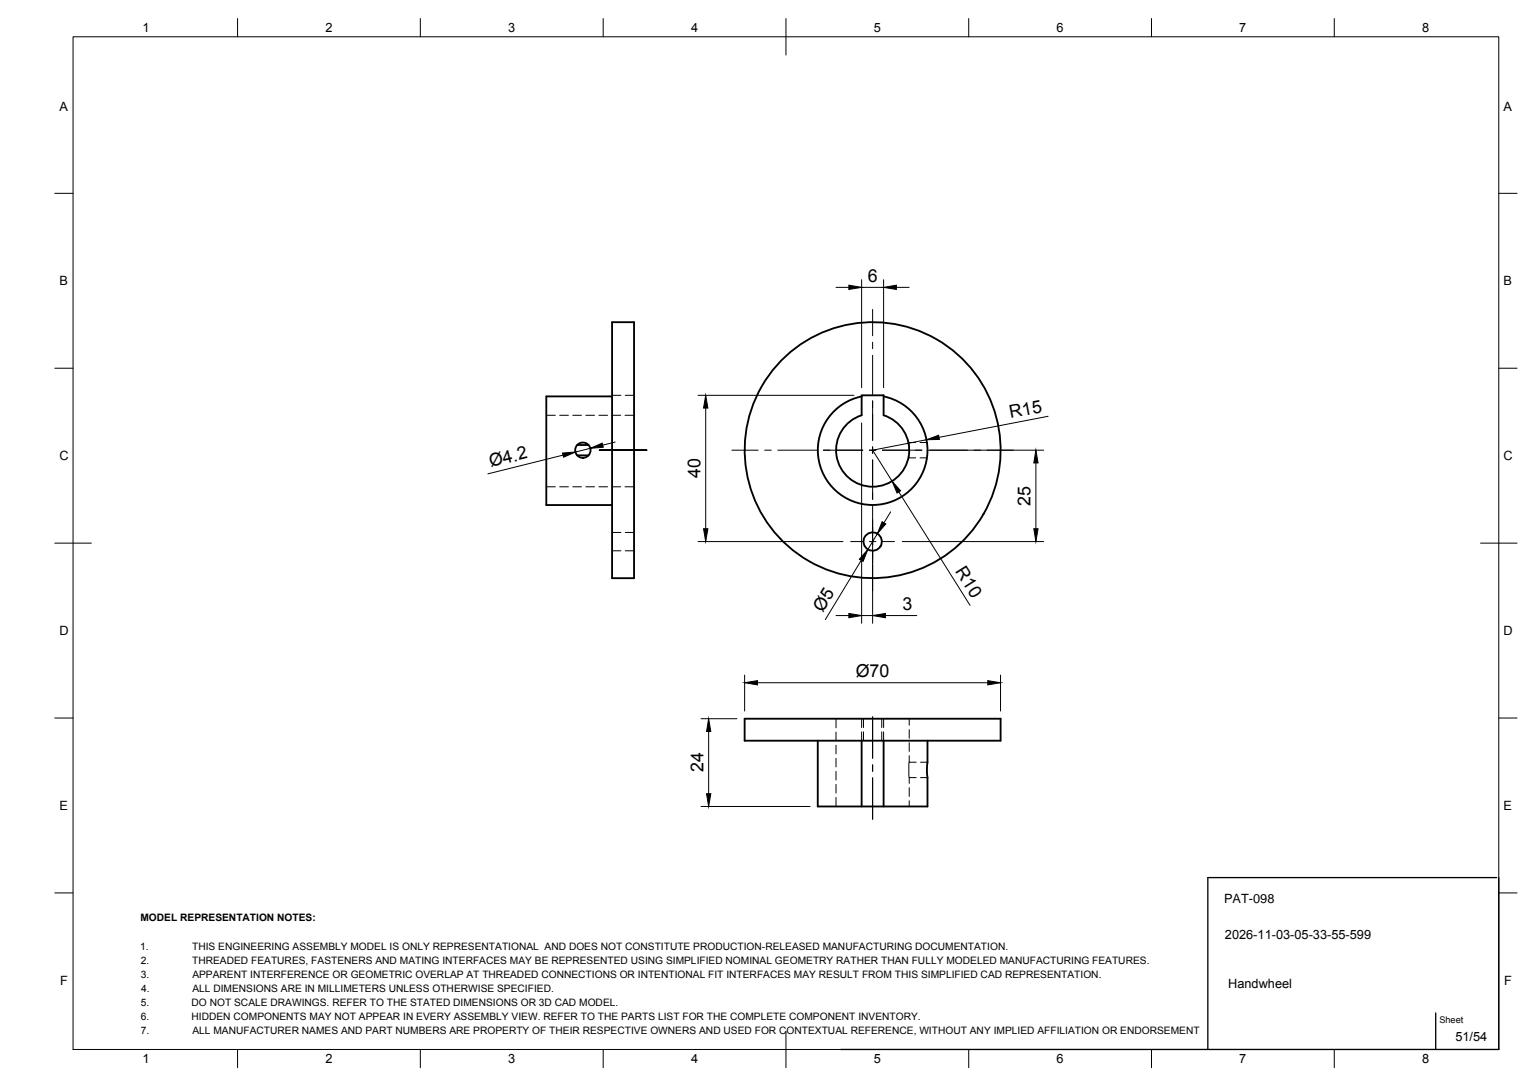
ISO-10303-21;
HEADER;
/* Generated by software containing ST-Developer
 * from STEP Tools, Inc. (www.steptools.com) 
 */

FILE_DESCRIPTION(
/* description */ ('Spring compression tester'),
/* implementation_level */ '2;1');

FILE_NAME(
/* name */ 'Handwheel.step',
/* time_stamp */ '2026-10-28T03:24:11-07:00',
/* author */ (''),
/* organization */ (''),
/* preprocessor_version */ 'ST-DEVELOPER v20.2',
/* originating_system */ 'Autodesk Translation Framework v15.17.0.0',
/* authorisation */ '');

FILE_SCHEMA (('AUTOMOTIVE_DESIGN { 1 0 10303 214 3 1 1 }'));
ENDSEC;

DATA;
#10=MECHANICAL_DESIGN_GEOMETRIC_PRESENTATION_REPRESENTATION('',(#1172),#43521);
#892=B_SPLINE_CURVE_WITH_KNOTS('',3,(#43043,#43044,#43045,#43046,#43047,
#43048),.UNSPECIFIED.,.F.,.F.,(4,2,4),(0.803821788694078,0.872950991853625,
0.952307212900975),.UNSPECIFIED.);
#893=B_SPLINE_CURVE_WITH_KNOTS('',3,(#43051,#43052,#43053,#43054,#43055,
#43056,#43057,#43058,#43059,#43060),.UNSPECIFIED.,.F.,.F.,(4,2,2,2,4),(0.168950313426762,
0.238079516586309,0.317435737633658,0.396791958681008,0.465921161840561),
 .UNSPECIFIED.);
#894=B_SPLINE_CURVE_WITH_KNOTS('',3,(#43061,#43062,#43063,#43064,#43065,
#43066),.UNSPECIFIED.,.F.,.F.,(4,2,4),(0.952307212900975,1.03166343394832,
1.10079263710787),.UNSPECIFIED.);
#895=B_SPLINE_CURVE_WITH_KNOTS('',3,(#43070,#43071,#43072,#43073,#43074,
#43075,#43076,#43077,#43078,#43079),.UNSPECIFIED.,.F.,.F.,(4,2,2,2,4),(0.,
0.0792165807733642,0.158433161546728,0.237648697074572,0.316864232602417),
 .UNSPECIFIED.);
#896=B_SPLINE_CURVE_WITH_KNOTS('',3,(#43080,#43081,#43082,#43083,#43084,
#43085,#43086,#43087,#43088,#43089,#43090,#43091,#43092,#43093,#43094,#43095,
#43096,#43097,#43098,#43099,#43100,#43101,#43102,#43103,#43104,#43105),
 .UNSPECIFIED.,.F.,.F.,(4,2,2,2,2,2,2,2,2,2,2,2,4),(0.316864232602417,0.396079768130261,
0.475295303658105,0.554511884431469,0.633728465204833,0.712945045978197,
0.792161626751562,0.871377162279406,0.95059269780725,1.02980823333509,1.10902376886294,
1.1882403496363,1.26745693040967),.UNSPECIFIED.);
#1037=SHAPE_REPRESENTATION_RELATIONSHIP('SRR','None',#43854,#1097);
#1097=ADVANCED_BREP_SHAPE_REPRESENTATION('',(#1241),#43514);
#1172=STYLED_ITEM('',(#44195),#1241);
#1241=MANIFOLD_SOLID_BREP('Body1',#18615);
#1575=FACE_BOUND('',#4536,.T.);
#1576=FACE_BOUND('',#4537,.T.);
#1577=FACE_BOUND('',#4539,.T.);
#1578=FACE_BOUND('',#4540,.T.);
#1579=FACE_BOUND('',#4543,.T.);
#1580=FACE_BOUND('',#4545,.T.);
#2126=PLANE('',#21081);
#2127=PLANE('',#21085);
#2128=PLANE('',#21086);
#2129=PLANE('',#21087);
#2130=PLANE('',#21088);
#2131=PLANE('',#21089);
#2132=PLANE('',#21092);
#2133=PLANE('',#21100);
#3153=FACE_OUTER_BOUND('',#4528,.T.);
#3154=FACE_OUTER_BOUND('',#4529,.T.);
#3155=FACE_OUTER_BOUND('',#4530,.T.);
#3156=FACE_OUTER_BOUND('',#4531,.T.);
#3157=FACE_OUTER_BOUND('',#4532,.T.);
#3158=FACE_OUTER_BOUND('',#4533,.T.);
#3159=FACE_OUTER_BOUND('',#4534,.T.);
#3160=FACE_OUTER_BOUND('',#4535,.T.);
#3161=FACE_OUTER_BOUND('',#4538,.T.);
#3162=FACE_OUTER_BOUND('',#4541,.T.);
#3163=FACE_OUTER_BOUND('',#4542,.T.);
#3164=FACE_OUTER_BOUND('',#4544,.T.);
#3165=FACE_OUTER_BOUND('',#4546,.T.);
#4528=EDGE_LOOP('',(#16839,#16840,#16841,#16842));
#4529=EDGE_LOOP('',(#16843,#16844));
#4530=EDGE_LOOP('',(#16845,#16846,#16847,#16848,#16849,#16850,#16851,#16852,
#16853));
#4531=EDGE_LOOP('',(#16854,#16855));
#4532=EDGE_LOOP('',(#16856,#16857,#16858,#16859,#16860,#16861));
#4533=EDGE_LOOP('',(#16862,#16863,#16864,#16865));
#4534=EDGE_LOOP('',(#16866,#16867,#16868,#16869,#16870,#16871));
#4535=EDGE_LOOP('',(#16872));
#4536=EDGE_LOOP('',(#16873));
#4537=EDGE_LOOP('',(#16874,#16875,#16876,#16877));
#4538=EDGE_LOOP('',(#16878));
#4539=EDGE_LOOP('',(#16879));
#4540=EDGE_LOOP('',(#16880,#16881,#16882,#16883));
#4541=EDGE_LOOP('',(#16884,#16885,#16886,#16887));
#4542=EDGE_LOOP('',(#16888,#16889,#16890,#16891));
#4543=EDGE_LOOP('',(#16892,#16893,#16894,#16895,#16896));
#4544=EDGE_LOOP('',(#16897,#16898,#16899,#16900));
#4545=EDGE_LOOP('',(#16901,#16902));
#4546=EDGE_LOOP('',(#16903,#16904,#16905,#16906));
#5944=LINE('',#43033,#7376);
#5945=LINE('',#43038,#7377);
#5946=LINE('',#43068,#7378);
#5947=LINE('',#43107,#7379);
#5948=LINE('',#43111,#7380);
#5949=LINE('',#43113,#7381);
#5950=LINE('',#43115,#7382);
#5951=LINE('',#43117,#7383);
#5952=LINE('',#43119,#7384);
#5953=LINE('',#43120,#7385);
#5954=LINE('',#43123,#7386);
#5955=LINE('',#43125,#7387);
#5956=LINE('',#43126,#7388);
#5957=LINE('',#43129,#7389);
#5958=LINE('',#43131,#7390);
#5959=LINE('',#43133,#7391);
#5960=LINE('',#43135,#7392);
#5961=LINE('',#43136,#7393);
#5962=LINE('',#43146,#7394);
#7376=VECTOR('',#26126,0.25);
#7377=VECTOR('',#26131,1.);
#7378=VECTOR('',#26138,0.210000000000001);
#7379=VECTOR('',#26141,1.);
#7380=VECTOR('',#26144,1.);
#7381=VECTOR('',#26145,1.);
#7382=VECTOR('',#26146,1.);
#7383=VECTOR('',#26147,1.);
#7384=VECTOR('',#26148,1.);
#7385=VECTOR('',#26149,1.);
#7386=VECTOR('',#26152,1.);
#7387=VECTOR('',#26153,1.);
#7388=VECTOR('',#26154,1.);
#7389=VECTOR('',#26157,1.);
#7390=VECTOR('',#26158,1.);
#7391=VECTOR('',#26159,1.);
#7392=VECTOR('',#26160,1.);
#7393=VECTOR('',#26161,1.);
#7394=VECTOR('',#26176,3.5);
#8102=CIRCLE('',#21079,0.25);
#8103=CIRCLE('',#21080,0.25);
#8104=CIRCLE('',#21082,0.210000000000001);
#8105=CIRCLE('',#21084,0.210000000000001);
#8106=CIRCLE('',#21090,3.5);
#8107=CIRCLE('',#21091,1.);
#8108=CIRCLE('',#21093,3.5);
#8109=CIRCLE('',#21094,1.5);
#8110=CIRCLE('',#21097,1.);
#8111=CIRCLE('',#21099,1.5);
#9686=VERTEX_POINT('',#43030);
#9687=VERTEX_POINT('',#43032);
#9688=VERTEX_POINT('',#43036);
#9689=VERTEX_POINT('',#43037);
#9690=VERTEX_POINT('',#43041);
#9691=VERTEX_POINT('',#43042);
#9692=VERTEX_POINT('',#43049);
#9693=VERTEX_POINT('',#43067);
#9694=VERTEX_POINT('',#43069);
#9695=VERTEX_POINT('',#43109);
#9696=VERTEX_POINT('',#43110);
#9697=VERTEX_POINT('',#43112);
#9698=VERTEX_POINT('',#43114);
#9699=VERTEX_POINT('',#43116);
#9700=VERTEX_POINT('',#43118);
#9701=VERTEX_POINT('',#43122);
#9702=VERTEX_POINT('',#43124);
#9703=VERTEX_POINT('',#43128);
#9704=VERTEX_POINT('',#43130);
#9705=VERTEX_POINT('',#43132);
#9706=VERTEX_POINT('',#43134);
#9707=VERTEX_POINT('',#43138);
#9708=VERTEX_POINT('',#43142);
#12084=EDGE_CURVE('',#9686,#9686,#8102,.T.);
#12085=EDGE_CURVE('',#9686,#9687,#5944,.T.);
#12086=EDGE_CURVE('',#9687,#9687,#8103,.T.);
#12087=EDGE_CURVE('',#9688,#9689,#5945,.T.);
#12088=EDGE_CURVE('',#9688,#9689,#8104,.T.);
#12089=EDGE_CURVE('',#9690,#9691,#892,.T.);
#12090=EDGE_CURVE('',#9692,#9690,#8105,.T.);
#12091=EDGE_CURVE('',#9689,#9692,#893,.T.);
#12092=EDGE_CURVE('',#9691,#9688,#894,.T.);
#12093=EDGE_CURVE('',#9691,#9693,#5946,.T.);
#12094=EDGE_CURVE('',#9694,#9693,#895,.T.);
#12095=EDGE_CURVE('',#9693,#9694,#896,.T.);
#12096=EDGE_CURVE('',#9692,#9690,#5947,.T.);
#12097=EDGE_CURVE('',#9695,#9696,#5948,.T.);
#12098=EDGE_CURVE('',#9697,#9695,#5949,.T.);
#12099=EDGE_CURVE('',#9698,#9697,#5950,.T.);
#12100=EDGE_CURVE('',#9699,#9698,#5951,.T.);
#12101=EDGE_CURVE('',#9700,#9699,#5952,.T.);
#12102=EDGE_CURVE('',#9696,#9700,#5953,.T.);
#12103=EDGE_CURVE('',#9701,#9695,#5954,.T.);
#12104=EDGE_CURVE('',#9702,#9701,#5955,.T.);
#12105=EDGE_CURVE('',#9697,#9702,#5956,.T.);
#12106=EDGE_CURVE('',#9703,#9701,#5957,.T.);
#12107=EDGE_CURVE('',#9704,#9703,#5958,.T.);
#12108=EDGE_CURVE('',#9705,#9704,#5959,.T.);
#12109=EDGE_CURVE('',#9706,#9705,#5960,.T.);
#12110=EDGE_CURVE('',#9702,#9706,#5961,.T.);
#12111=EDGE_CURVE('',#9707,#9707,#8106,.T.);
#12112=EDGE_CURVE('',#9696,#9703,#8107,.T.);
#12113=EDGE_CURVE('',#9708,#9708,#8108,.T.);
#12114=EDGE_CURVE('',#9706,#9698,#8109,.T.);
#12115=EDGE_CURVE('',#9707,#9708,#5962,.T.);
#12116=EDGE_CURVE('',#9700,#9704,#8110,.T.);
#12117=EDGE_CURVE('',#9705,#9699,#8111,.T.);
#16839=ORIENTED_EDGE('',*,*,#12084,.F.);
#16840=ORIENTED_EDGE('',*,*,#12085,.T.);
#16841=ORIENTED_EDGE('',*,*,#12086,.F.);
#16842=ORIENTED_EDGE('',*,*,#12085,.F.);
#16843=ORIENTED_EDGE('',*,*,#12087,.F.);
#16844=ORIENTED_EDGE('',*,*,#12088,.T.);
#16845=ORIENTED_EDGE('',*,*,#12089,.F.);
#16846=ORIENTED_EDGE('',*,*,#12090,.F.);
#16847=ORIENTED_EDGE('',*,*,#12091,.F.);
#16848=ORIENTED_EDGE('',*,*,#12088,.F.);
#16849=ORIENTED_EDGE('',*,*,#12092,.F.);
#16850=ORIENTED_EDGE('',*,*,#12093,.T.);
#16851=ORIENTED_EDGE('',*,*,#12094,.F.);
#16852=ORIENTED_EDGE('',*,*,#12095,.F.);
#16853=ORIENTED_EDGE('',*,*,#12093,.F.);
#16854=ORIENTED_EDGE('',*,*,#12096,.F.);
#16855=ORIENTED_EDGE('',*,*,#12090,.T.);
#16856=ORIENTED_EDGE('',*,*,#12097,.F.);
#16857=ORIENTED_EDGE('',*,*,#12098,.F.);
#16858=ORIENTED_EDGE('',*,*,#12099,.F.);
#16859=ORIENTED_EDGE('',*,*,#12100,.F.);
#16860=ORIENTED_EDGE('',*,*,#12101,.F.);
#16861=ORIENTED_EDGE('',*,*,#12102,.F.);
#16862=ORIENTED_EDGE('',*,*,#12103,.F.);
#16863=ORIENTED_EDGE('',*,*,#12104,.F.);
#16864=ORIENTED_EDGE('',*,*,#12105,.F.);
#16865=ORIENTED_EDGE('',*,*,#12098,.T.);
#16866=ORIENTED_EDGE('',*,*,#12106,.F.);
#16867=ORIENTED_EDGE('',*,*,#12107,.F.);
#16868=ORIENTED_EDGE('',*,*,#12108,.F.);
#16869=ORIENTED_EDGE('',*,*,#12109,.F.);
#16870=ORIENTED_EDGE('',*,*,#12110,.F.);
#16871=ORIENTED_EDGE('',*,*,#12104,.T.);
#16872=ORIENTED_EDGE('',*,*,#12111,.T.);
#16873=ORIENTED_EDGE('',*,*,#12086,.T.);
#16874=ORIENTED_EDGE('',*,*,#12106,.T.);
#16875=ORIENTED_EDGE('',*,*,#12103,.T.);
#16876=ORIENTED_EDGE('',*,*,#12097,.T.);
#16877=ORIENTED_EDGE('',*,*,#12112,.T.);
#16878=ORIENTED_EDGE('',*,*,#12113,.F.);
#16879=ORIENTED_EDGE('',*,*,#12084,.T.);
#16880=ORIENTED_EDGE('',*,*,#12110,.T.);
#16881=ORIENTED_EDGE('',*,*,#12114,.T.);
#16882=ORIENTED_EDGE('',*,*,#12099,.T.);
#16883=ORIENTED_EDGE('',*,*,#12105,.T.);
#16884=ORIENTED_EDGE('',*,*,#12111,.F.);
#16885=ORIENTED_EDGE('',*,*,#12115,.T.);
#16886=ORIENTED_EDGE('',*,*,#12113,.T.);
#16887=ORIENTED_EDGE('',*,*,#12115,.F.);
#16888=ORIENTED_EDGE('',*,*,#12107,.T.);
#16889=ORIENTED_EDGE('',*,*,#12112,.F.);
#16890=ORIENTED_EDGE('',*,*,#12102,.T.);
#16891=ORIENTED_EDGE('',*,*,#12116,.T.);
#16892=ORIENTED_EDGE('',*,*,#12091,.T.);
#16893=ORIENTED_EDGE('',*,*,#12096,.T.);
#16894=ORIENTED_EDGE('',*,*,#12089,.T.);
#16895=ORIENTED_EDGE('',*,*,#12092,.T.);
#16896=ORIENTED_EDGE('',*,*,#12087,.T.);
#16897=ORIENTED_EDGE('',*,*,#12109,.T.);
#16898=ORIENTED_EDGE('',*,*,#12117,.T.);
#16899=ORIENTED_EDGE('',*,*,#12100,.T.);
#16900=ORIENTED_EDGE('',*,*,#12114,.F.);
#16901=ORIENTED_EDGE('',*,*,#12094,.T.);
#16902=ORIENTED_EDGE('',*,*,#12095,.T.);
#16903=ORIENTED_EDGE('',*,*,#12108,.T.);
#16904=ORIENTED_EDGE('',*,*,#12116,.F.);
#16905=ORIENTED_EDGE('',*,*,#12101,.T.);
#16906=ORIENTED_EDGE('',*,*,#12117,.F.);
#17480=CYLINDRICAL_SURFACE('',#21078,0.25);
#17481=CYLINDRICAL_SURFACE('',#21083,0.210000000000001);
#17482=CYLINDRICAL_SURFACE('',#21095,3.5);
#17483=CYLINDRICAL_SURFACE('',#21096,1.);
#17484=CYLINDRICAL_SURFACE('',#21098,1.5);
#18477=ADVANCED_FACE('',(#3153),#17480,.F.);
#18478=ADVANCED_FACE('',(#3154),#2126,.T.);
#18479=ADVANCED_FACE('',(#3155),#17481,.F.);
#18480=ADVANCED_FACE('',(#3156),#2127,.T.);
#18481=ADVANCED_FACE('',(#3157),#2128,.F.);
#18482=ADVANCED_FACE('',(#3158),#2129,.F.);
#18483=ADVANCED_FACE('',(#3159),#2130,.F.);
#18484=ADVANCED_FACE('',(#3160,#1575,#1576),#2131,.T.);
#18485=ADVANCED_FACE('',(#3161,#1577,#1578),#2132,.F.);
#18486=ADVANCED_FACE('',(#3162),#17482,.T.);
#18487=ADVANCED_FACE('',(#3163,#1579),#17483,.F.);
#18488=ADVANCED_FACE('',(#3164,#1580),#17484,.T.);
#18489=ADVANCED_FACE('',(#3165),#2133,.F.);
#18615=CLOSED_SHELL('',(#18477,#18478,#18479,#18480,#18481,#18482,#18483,
#18484,#18485,#18486,#18487,#18488,#18489));
#21077=AXIS2_PLACEMENT_3D('',#43028,#26120,#26121);
#21078=AXIS2_PLACEMENT_3D('',#43029,#26122,#26123);
#21079=AXIS2_PLACEMENT_3D('',#43031,#26124,#26125);
#21080=AXIS2_PLACEMENT_3D('',#43034,#26127,#26128);
#21081=AXIS2_PLACEMENT_3D('',#43035,#26129,#26130);
#21082=AXIS2_PLACEMENT_3D('',#43039,#26132,#26133);
#21083=AXIS2_PLACEMENT_3D('',#43040,#26134,#26135);
#21084=AXIS2_PLACEMENT_3D('',#43050,#26136,#26137);
#21085=AXIS2_PLACEMENT_3D('',#43106,#26139,#26140);
#21086=AXIS2_PLACEMENT_3D('',#43108,#26142,#26143);
#21087=AXIS2_PLACEMENT_3D('',#43121,#26150,#26151);
#21088=AXIS2_PLACEMENT_3D('',#43127,#26155,#26156);
#21089=AXIS2_PLACEMENT_3D('',#43137,#26162,#26163);
#21090=AXIS2_PLACEMENT_3D('',#43139,#26164,#26165);
#21091=AXIS2_PLACEMENT_3D('',#43140,#26166,#26167);
#21092=AXIS2_PLACEMENT_3D('',#43141,#26168,#26169);
#21093=AXIS2_PLACEMENT_3D('',#43143,#26170,#26171);
#21094=AXIS2_PLACEMENT_3D('',#43144,#26172,#26173);
#21095=AXIS2_PLACEMENT_3D('',#43145,#26174,#26175);
#21096=AXIS2_PLACEMENT_3D('',#43147,#26177,#26178);
#21097=AXIS2_PLACEMENT_3D('',#43148,#26179,#26180);
#21098=AXIS2_PLACEMENT_3D('',#43149,#26181,#26182);
#21099=AXIS2_PLACEMENT_3D('',#43150,#26183,#26184);
#21100=AXIS2_PLACEMENT_3D('',#43151,#26185,#26186);
#26120=DIRECTION('axis',(0.,0.,1.));
#26121=DIRECTION('refdir',(1.,0.,0.));
#26122=DIRECTION('center_axis',(1.,0.,0.));
#26123=DIRECTION('ref_axis',(0.,0.,-1.));
#26124=DIRECTION('center_axis',(1.,0.,0.));
#26125=DIRECTION('ref_axis',(0.,0.,-1.));
#26126=DIRECTION('',(1.,0.,0.));
#26127=DIRECTION('center_axis',(-1.,0.,0.));
#26128=DIRECTION('ref_axis',(0.,0.,-1.));
#26129=DIRECTION('center_axis',(0.,1.,0.));
#26130=DIRECTION('ref_axis',(1.,0.,0.));
#26131=DIRECTION('',(1.,0.,0.));
#26132=DIRECTION('center_axis',(0.,1.,0.));
#26133=DIRECTION('ref_axis',(1.,0.,0.));
#26134=DIRECTION('center_axis',(0.,1.,0.));
#26135=DIRECTION('ref_axis',(1.,0.,0.));
#26136=DIRECTION('center_axis',(0.,1.,0.));
#26137=DIRECTION('ref_axis',(1.,0.,0.));
#26138=DIRECTION('',(0.,1.,0.));
#26139=DIRECTION('center_axis',(0.,1.,0.));
#26140=DIRECTION('ref_axis',(1.,0.,0.));
#26141=DIRECTION('',(-1.,0.,0.));
#26142=DIRECTION('center_axis',(0.,-1.,0.));
#26143=DIRECTION('ref_axis',(0.,0.,-1.));
#26144=DIRECTION('',(0.,0.,1.));
#26145=DIRECTION('',(1.,0.,0.));
#26146=DIRECTION('',(0.,0.,-1.));
#26147=DIRECTION('',(1.,0.,0.));
#26148=DIRECTION('',(0.,0.,-1.));
#26149=DIRECTION('',(-1.,0.,0.));
#26150=DIRECTION('center_axis',(0.,0.,-1.));
#26151=DIRECTION('ref_axis',(0.,1.,0.));
#26152=DIRECTION('',(0.,-1.,0.));
#26153=DIRECTION('',(1.,0.,0.));
#26154=DIRECTION('',(0.,1.,0.));
#26155=DIRECTION('center_axis',(0.,1.,0.));
#26156=DIRECTION('ref_axis',(0.,0.,1.));
#26157=DIRECTION('',(0.,0.,-1.));
#26158=DIRECTION('',(1.,0.,0.));
#26159=DIRECTION('',(0.,0.,1.));
#26160=DIRECTION('',(-1.,0.,0.));
#26161=DIRECTION('',(0.,0.,1.));
#26162=DIRECTION('center_axis',(1.,0.,0.));
#26163=DIRECTION('ref_axis',(0.,0.,-1.));
#26164=DIRECTION('center_axis',(1.,0.,0.));
#26165=DIRECTION('ref_axis',(0.,0.,-1.));
#26166=DIRECTION('center_axis',(-1.,0.,0.));
#26167=DIRECTION('ref_axis',(0.,0.,-1.));
#26168=DIRECTION('center_axis',(1.,0.,0.));
#26169=DIRECTION('ref_axis',(0.,0.,-1.));
#26170=DIRECTION('center_axis',(1.,0.,0.));
#26171=DIRECTION('ref_axis',(0.,0.,-1.));
#26172=DIRECTION('center_axis',(1.,0.,0.));
#26173=DIRECTION('ref_axis',(0.,0.,-1.));
#26174=DIRECTION('center_axis',(1.,0.,0.));
#26175=DIRECTION('ref_axis',(0.,0.,-1.));
#26176=DIRECTION('',(-1.,0.,0.));
#26177=DIRECTION('center_axis',(1.,0.,0.));
#26178=DIRECTION('ref_axis',(0.,1.22464679914735E-16,1.));
#26179=DIRECTION('center_axis',(-1.,0.,0.));
#26180=DIRECTION('ref_axis',(0.,0.,-1.));
#26181=DIRECTION('center_axis',(1.,0.,0.));
#26182=DIRECTION('ref_axis',(0.,1.22464679914735E-16,1.));
#26183=DIRECTION('center_axis',(1.,0.,0.));
#26184=DIRECTION('ref_axis',(0.,0.,-1.));
#26185=DIRECTION('center_axis',(1.,0.,0.));
#26186=DIRECTION('ref_axis',(0.,0.,-1.));
#43028=CARTESIAN_POINT('',(0.,0.,0.));
#43029=CARTESIAN_POINT('Origin',(28.7,0.,6.5));
#43030=CARTESIAN_POINT('',(28.8,-3.06161699786838E-17,6.75));
#43031=CARTESIAN_POINT('Origin',(28.8,0.,6.5));
#43032=CARTESIAN_POINT('',(29.4,3.06161699786838E-17,6.75));
#43033=CARTESIAN_POINT('',(28.7,-3.06161699786838E-17,6.75));
#43034=CARTESIAN_POINT('Origin',(29.4,0.,6.5));
#43035=CARTESIAN_POINT('Origin',(28.,0.99,4.));
#43036=CARTESIAN_POINT('',(27.844436508139,0.99,4.14106735979666));
#43037=CARTESIAN_POINT('',(28.155563491861,0.99,4.14106735979666));
#43038=CARTESIAN_POINT('',(27.,0.99,4.14106735979666));
#43039=CARTESIAN_POINT('Origin',(28.,0.99,4.));
#43040=CARTESIAN_POINT('Origin',(28.,0.99,4.));
#43041=CARTESIAN_POINT('',(27.844436508139,0.99,3.85893264020334));
#43042=CARTESIAN_POINT('',(27.79,1.,4.));
#43043=CARTESIAN_POINT('Ctrl Pts',(27.844436508139,0.99,3.85893264020334));
#43044=CARTESIAN_POINT('Ctrl Pts',(27.8287948476368,0.992457849824465,3.87618164330178));
#43045=CARTESIAN_POINT('Ctrl Pts',(27.815375956669,0.994938193049464,3.8970013568903));
#43046=CARTESIAN_POINT('Ctrl Pts',(27.7953025362756,0.998844492372413,3.94538588560165));
#43047=CARTESIAN_POINT('Ctrl Pts',(27.79,1.,3.97354792631755));
#43048=CARTESIAN_POINT('Ctrl Pts',(27.79,1.,4.));
#43049=CARTESIAN_POINT('',(28.155563491861,0.99,3.85893264020334));
#43050=CARTESIAN_POINT('Origin',(28.,0.99,4.));
#43051=CARTESIAN_POINT('Ctrl Pts',(28.155563491861,0.99,4.14106735979666));
#43052=CARTESIAN_POINT('Ctrl Pts',(28.1712051523632,0.992457849824465,4.12381835669823));
#43053=CARTESIAN_POINT('Ctrl Pts',(28.184624043331,0.994938193049464,4.1029986431097));
#43054=CARTESIAN_POINT('Ctrl Pts',(28.2046974637244,0.998844492372413,4.05461411439835));
#43055=CARTESIAN_POINT('Ctrl Pts',(28.21,1.,4.02645207368245));
#43056=CARTESIAN_POINT('Ctrl Pts',(28.21,1.,3.97354792631755));
#43057=CARTESIAN_POINT('Ctrl Pts',(28.2046974637244,0.998844492372413,3.94538588560165));
#43058=CARTESIAN_POINT('Ctrl Pts',(28.184624043331,0.994938193049464,3.8970013568903));
#43059=CARTESIAN_POINT('Ctrl Pts',(28.1712051523632,0.992457849824465,3.87618164330178));
#43060=CARTESIAN_POINT('Ctrl Pts',(28.155563491861,0.99,3.85893264020334));
#43061=CARTESIAN_POINT('Ctrl Pts',(27.79,1.,4.));
#43062=CARTESIAN_POINT('Ctrl Pts',(27.79,1.,4.02645207368245));
#43063=CARTESIAN_POINT('Ctrl Pts',(27.7953025362756,0.998844492372413,4.05461411439835));
#43064=CARTESIAN_POINT('Ctrl Pts',(27.815375956669,0.994938193049464,4.1029986431097));
#43065=CARTESIAN_POINT('Ctrl Pts',(27.8287948476368,0.992457849824465,4.12381835669823));
#43066=CARTESIAN_POINT('Ctrl Pts',(27.844436508139,0.99,4.14106735979666));
#43067=CARTESIAN_POINT('',(27.79,1.5,4.));
#43068=CARTESIAN_POINT('',(27.79,0.99,4.));
#43069=CARTESIAN_POINT('',(28.,1.48522725533839,4.21));
#43070=CARTESIAN_POINT('Ctrl Pts',(28.,1.48522725533839,4.21));
#43071=CARTESIAN_POINT('Ctrl Pts',(27.9735944730755,1.48522725533839,4.21));
#43072=CARTESIAN_POINT('Ctrl Pts',(27.9454529259093,1.48600415954412,4.20471573726959));
#43073=CARTESIAN_POINT('Ctrl Pts',(27.8937237310949,1.48880073282317,4.18327376303633));
#43074=CARTESIAN_POINT('Ctrl Pts',(27.870133075872,1.49077897157582,4.16711792397039));
#43075=CARTESIAN_POINT('Ctrl Pts',(27.832882321789,1.49448481141327,4.12986716988737));
#43076=CARTESIAN_POINT('Ctrl Pts',(27.8167262899986,1.49645455657129,4.10627640830576));
#43077=CARTESIAN_POINT('Ctrl Pts',(27.7952841751738,1.49923165515646,4.0545468514059));
#43078=CARTESIAN_POINT('Ctrl Pts',(27.79,1.5,4.02640517850928));
#43079=CARTESIAN_POINT('Ctrl Pts',(27.79,1.5,4.));
#43080=CARTESIAN_POINT('Ctrl Pts',(27.79,1.5,4.));
#43081=CARTESIAN_POINT('Ctrl Pts',(27.79,1.5,3.97359482149072));
#43082=CARTESIAN_POINT('Ctrl Pts',(27.7952841751738,1.49923165515646,3.9454531485941));
#43083=CARTESIAN_POINT('Ctrl Pts',(27.8167262899986,1.49645455657129,3.89372359169424));
#43084=CARTESIAN_POINT('Ctrl Pts',(27.832882321789,1.49448481141327,3.87013283011263));
#43085=CARTESIAN_POINT('Ctrl Pts',(27.870133075872,1.49077897157582,3.83288207602961));
#43086=CARTESIAN_POINT('Ctrl Pts',(27.8937237310949,1.48880073282317,3.81672623696367));
#43087=CARTESIAN_POINT('Ctrl Pts',(27.9454529259093,1.48600415954412,3.7952842627304));
#43088=CARTESIAN_POINT('Ctrl Pts',(27.9735944730755,1.48522725533839,3.79));
#43089=CARTESIAN_POINT('Ctrl Pts',(28.0264055269245,1.48522725533839,3.79));
#43090=CARTESIAN_POINT('Ctrl Pts',(28.0545470740907,1.48600415954412,3.7952842627304));
#43091=CARTESIAN_POINT('Ctrl Pts',(28.1062762689051,1.48880073282317,3.81672623696367));
#43092=CARTESIAN_POINT('Ctrl Pts',(28.129866924128,1.49077897157582,3.83288207602961));
#43093=CARTESIAN_POINT('Ctrl Pts',(28.167117678211,1.49448481141327,3.87013283011263));
#43094=CARTESIAN_POINT('Ctrl Pts',(28.1832737100014,1.49645455657129,3.89372359169424));
#43095=CARTESIAN_POINT('Ctrl Pts',(28.2047158248262,1.49923165515646,3.9454531485941));
#43096=CARTESIAN_POINT('Ctrl Pts',(28.21,1.5,3.97359482149072));
#43097=CARTESIAN_POINT('Ctrl Pts',(28.21,1.5,4.02640517850928));
#43098=CARTESIAN_POINT('Ctrl Pts',(28.2047158248262,1.49923165515646,4.0545468514059));
#43099=CARTESIAN_POINT('Ctrl Pts',(28.1832737100014,1.49645455657129,4.10627640830576));
#43100=CARTESIAN_POINT('Ctrl Pts',(28.167117678211,1.49448481141327,4.12986716988737));
#43101=CARTESIAN_POINT('Ctrl Pts',(28.129866924128,1.49077897157582,4.16711792397039));
#43102=CARTESIAN_POINT('Ctrl Pts',(28.1062762689051,1.48880073282317,4.18327376303633));
#43103=CARTESIAN_POINT('Ctrl Pts',(28.0545470740907,1.48600415954412,4.2047157372696));
#43104=CARTESIAN_POINT('Ctrl Pts',(28.0264055269245,1.48522725533839,4.21));
#43105=CARTESIAN_POINT('Ctrl Pts',(28.,1.48522725533839,4.21));
#43106=CARTESIAN_POINT('Origin',(28.,0.99,4.));
#43107=CARTESIAN_POINT('',(27.,0.99,3.85893264020334));
#43108=CARTESIAN_POINT('Origin',(26.9,-0.3,4.));
#43109=CARTESIAN_POINT('',(29.4,-0.3,2.5));
#43110=CARTESIAN_POINT('',(29.4,-0.3,3.04606079858305));
#43111=CARTESIAN_POINT('',(29.4,-0.3,4.));
#43112=CARTESIAN_POINT('',(28.8,-0.3,2.5));
#43113=CARTESIAN_POINT('',(26.9,-0.3,2.5));
#43114=CARTESIAN_POINT('',(28.8,-0.3,2.53030615433009));
#43115=CARTESIAN_POINT('',(28.8,-0.3,4.));
#43116=CARTESIAN_POINT('',(27.,-0.3,2.53030615433009));
#43117=CARTESIAN_POINT('',(27.,-0.3,2.53030615433009));
#43118=CARTESIAN_POINT('',(27.,-0.3,3.04606079858305));
#43119=CARTESIAN_POINT('',(27.,-0.3,4.));
#43120=CARTESIAN_POINT('',(27.,-0.3,3.04606079858305));
#43121=CARTESIAN_POINT('Origin',(26.9,-0.3,2.5));
#43122=CARTESIAN_POINT('',(29.4,0.3,2.5));
#43123=CARTESIAN_POINT('',(29.4,-0.15,2.5));
#43124=CARTESIAN_POINT('',(28.8,0.3,2.5));
#43125=CARTESIAN_POINT('',(26.9,0.3,2.5));
#43126=CARTESIAN_POINT('',(28.8,-0.15,2.5));
#43127=CARTESIAN_POINT('Origin',(26.9,0.3,2.5));
#43128=CARTESIAN_POINT('',(29.4,0.3,3.04606079858305));
#43129=CARTESIAN_POINT('',(29.4,0.3,3.25));
#43130=CARTESIAN_POINT('',(27.,0.3,3.04606079858305));
#43131=CARTESIAN_POINT('',(27.,0.3,3.04606079858305));
#43132=CARTESIAN_POINT('',(27.,0.3,2.53030615433009));
#43133=CARTESIAN_POINT('',(27.,0.3,3.25));
#43134=CARTESIAN_POINT('',(28.8,0.3,2.53030615433009));
#43135=CARTESIAN_POINT('',(27.,0.3,2.53030615433009));
#43136=CARTESIAN_POINT('',(28.8,0.3,3.25));
#43137=CARTESIAN_POINT('Origin',(29.4,0.,4.));
#43138=CARTESIAN_POINT('',(29.4,-4.28626379701574E-16,7.5));
#43139=CARTESIAN_POINT('Origin',(29.4,0.,4.));
#43140=CARTESIAN_POINT('Origin',(29.4,0.,4.));
#43141=CARTESIAN_POINT('Origin',(28.8,0.,4.));
#43142=CARTESIAN_POINT('',(28.8,-4.28626379701574E-16,7.5));
#43143=CARTESIAN_POINT('Origin',(28.8,0.,4.));
#43144=CARTESIAN_POINT('Origin',(28.8,0.,4.));
#43145=CARTESIAN_POINT('Origin',(28.8,0.,4.));
#43146=CARTESIAN_POINT('',(28.8,-4.28626379701574E-16,7.5));
#43147=CARTESIAN_POINT('Origin',(27.,0.,4.));
#43148=CARTESIAN_POINT('Origin',(27.,0.,4.));
#43149=CARTESIAN_POINT('Origin',(27.,0.,4.));
#43150=CARTESIAN_POINT('Origin',(27.,0.,4.));
#43151=CARTESIAN_POINT('Origin',(27.,0.,4.));
#43446=UNCERTAINTY_MEASURE_WITH_UNIT(LENGTH_MEASURE(0.001),#43522,
'DISTANCE_ACCURACY_VALUE',
'Maximum model space distance between geometric entities at asserted c
onnectivities');
#43453=UNCERTAINTY_MEASURE_WITH_UNIT(LENGTH_MEASURE(0.001),#43522,
'DISTANCE_ACCURACY_VALUE',
'Maximum model space distance between geometric entities at asserted c
onnectivities');
#43514=(
GEOMETRIC_REPRESENTATION_CONTEXT(3)
GLOBAL_UNCERTAINTY_ASSIGNED_CONTEXT((#43446))
GLOBAL_UNIT_ASSIGNED_CONTEXT((#43522,#43524,#43525))
REPRESENTATION_CONTEXT('','3D')
);
#43521=(
GEOMETRIC_REPRESENTATION_CONTEXT(3)
GLOBAL_UNCERTAINTY_ASSIGNED_CONTEXT((#43453))
GLOBAL_UNIT_ASSIGNED_CONTEXT((#43522,#43524,#43525))
REPRESENTATION_CONTEXT('','3D')
);
#43522=(
LENGTH_UNIT()
NAMED_UNIT(*)
SI_UNIT(.CENTI.,.METRE.)
);
#43524=(
NAMED_UNIT(*)
PLANE_ANGLE_UNIT()
SI_UNIT($,.RADIAN.)
);
#43525=(
NAMED_UNIT(*)
SI_UNIT($,.STERADIAN.)
SOLID_ANGLE_UNIT()
);
#43586=SHAPE_DEFINITION_REPRESENTATION(#43773,#43854);
#43773=PRODUCT_DEFINITION_SHAPE('',$,#43922);
#43854=SHAPE_REPRESENTATION('',(#21077),#43514);
#43861=PRODUCT_DEFINITION_CONTEXT('part definition',#44064,'design');
#43922=PRODUCT_DEFINITION('Handwheel','Handwheel',#43989,#43861);
#43989=PRODUCT_DEFINITION_FORMATION('',$,#44126);
#44064=APPLICATION_CONTEXT(
'Core Data for Automotive Mechanical Design Process');
#44065=PRODUCT_CONTEXT('part definition',#44064,'mechanical');
#44126=PRODUCT('Handwheel','Handwheel','Handwheel',(#44065));
#44189=COLOUR_RGB('Sky Blue',0.24,0.69,0.87);
#44190=FILL_AREA_STYLE_COLOUR('',#44189);
#44191=FILL_AREA_STYLE('',(#44190));
#44192=SURFACE_STYLE_FILL_AREA(#44191);
#44193=SURFACE_SIDE_STYLE('',(#44192));
#44194=SURFACE_STYLE_USAGE(.BOTH.,#44193);
#44195=PRESENTATION_STYLE_ASSIGNMENT((#44194));
ENDSEC;
END-ISO-10303-21;
